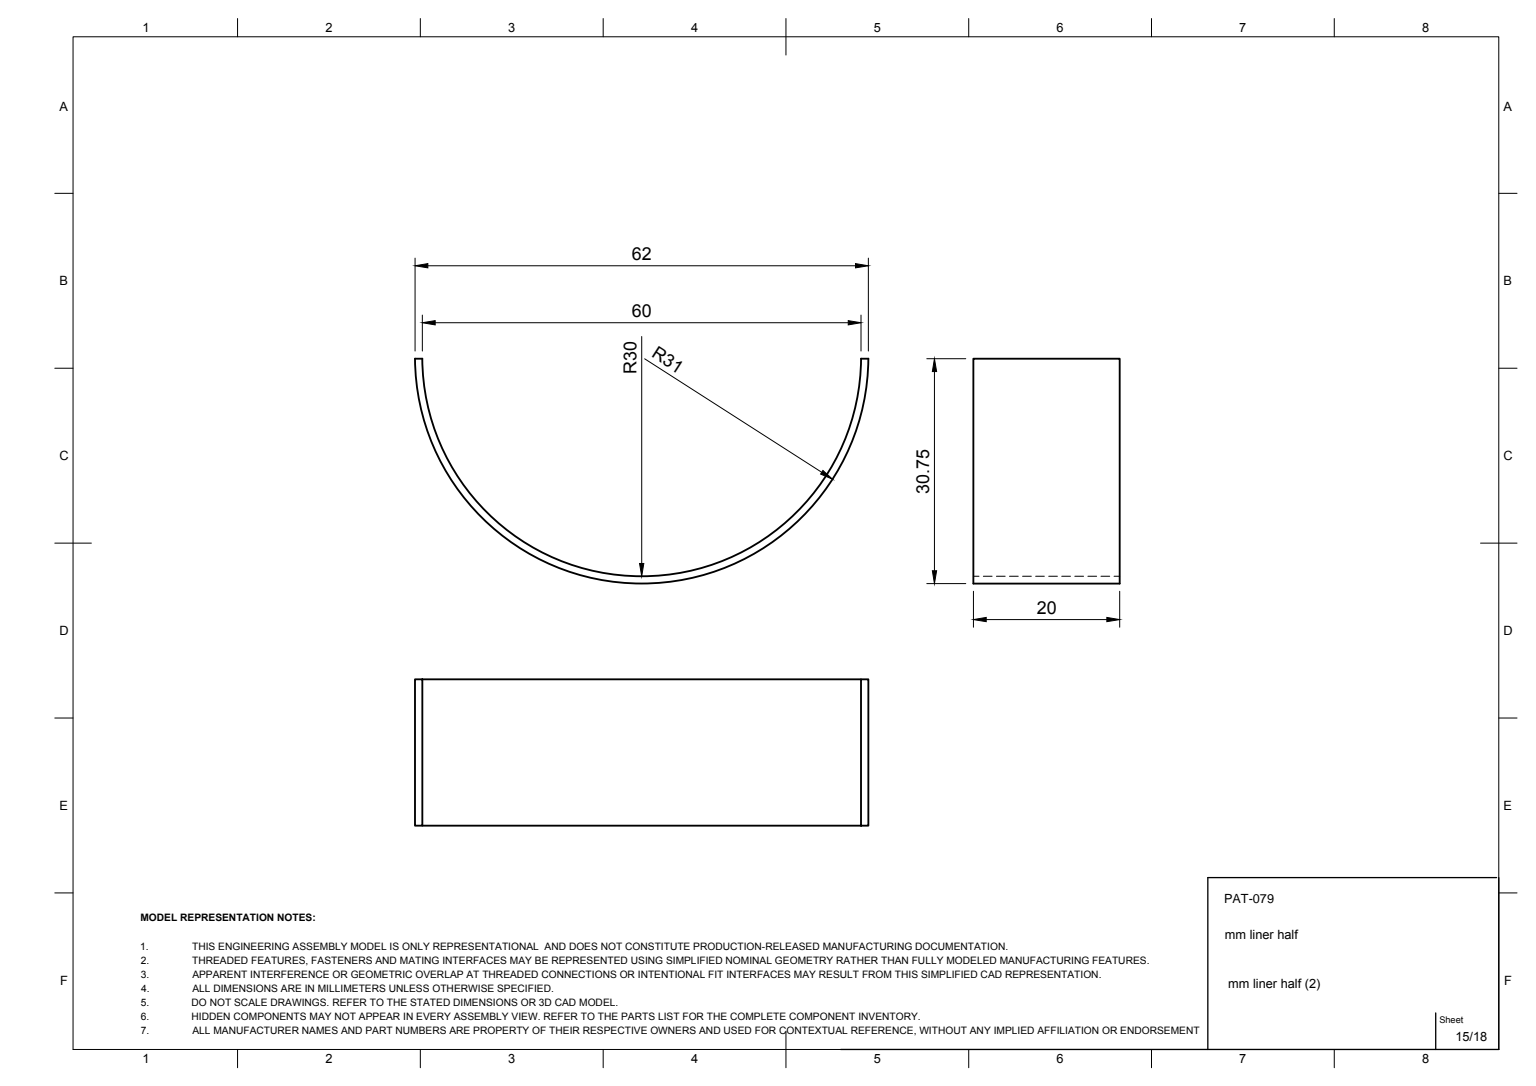
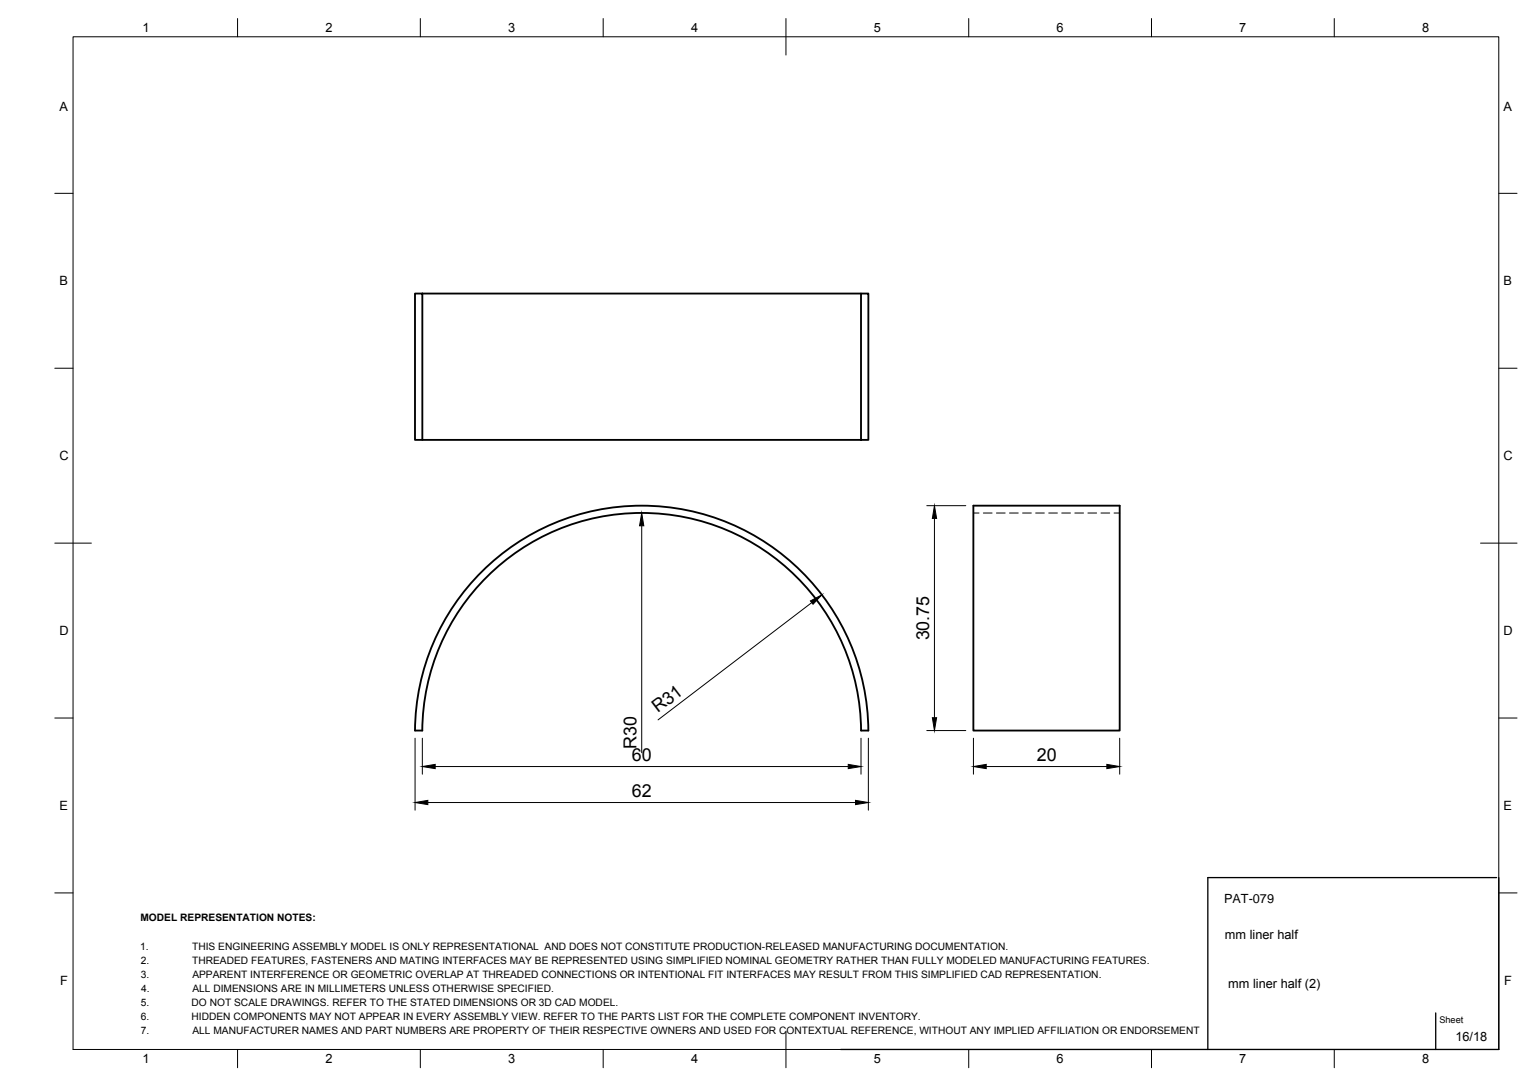
ISO-10303-21;
HEADER;
/* Generated by software containing ST-Developer
 * from STEP Tools, Inc. (www.steptools.com) 
 */

FILE_DESCRIPTION(
/* description */ ('Pipe clamp stand with threaded column'),
/* implementation_level */ '2;1');

FILE_NAME(
/* name */ 'mm liner half (2).step',
/* time_stamp */ '2026-10-27T10:55:48-07:00',
/* author */ (''),
/* organization */ (''),
/* preprocessor_version */ 'ST-DEVELOPER v20.2',
/* originating_system */ 'Autodesk Translation Framework v15.17.0.0',
/* authorisation */ '');

FILE_SCHEMA (('AUTOMOTIVE_DESIGN { 1 0 10303 214 3 1 1 }'));
ENDSEC;

DATA;
#10=MECHANICAL_DESIGN_GEOMETRIC_PRESENTATION_REPRESENTATION('',(#759),#34433);
#707=SHAPE_REPRESENTATION_RELATIONSHIP('SRR','None',#34549,#729);
#729=ADVANCED_BREP_SHAPE_REPRESENTATION('',(#789),#34417);
#759=STYLED_ITEM('',(#34736),#789);
#789=MANIFOLD_SOLID_BREP('Body1',#8786);
#959=PLANE('',#9474);
#960=PLANE('',#9475);
#961=PLANE('',#9476);
#962=PLANE('',#9483);
#1378=FACE_OUTER_BOUND('',#1908,.T.);
#1379=FACE_OUTER_BOUND('',#1909,.T.);
#1380=FACE_OUTER_BOUND('',#1910,.T.);
#1381=FACE_OUTER_BOUND('',#1911,.T.);
#1382=FACE_OUTER_BOUND('',#1912,.T.);
#1383=FACE_OUTER_BOUND('',#1913,.T.);
#1908=EDGE_LOOP('',(#7283,#7284,#7285,#7286));
#1909=EDGE_LOOP('',(#7287,#7288,#7289,#7290));
#1910=EDGE_LOOP('',(#7291,#7292,#7293,#7294));
#1911=EDGE_LOOP('',(#7295,#7296,#7297,#7298));
#1912=EDGE_LOOP('',(#7299,#7300,#7301,#7302));
#1913=EDGE_LOOP('',(#7303,#7304,#7305,#7306));
#2491=LINE('',#28574,#3108);
#2492=LINE('',#28576,#3109);
#2493=LINE('',#28578,#3110);
#2494=LINE('',#28579,#3111);
#2495=LINE('',#28583,#3112);
#2496=LINE('',#28585,#3113);
#2497=LINE('',#28587,#3114);
#2498=LINE('',#28588,#3115);
#3108=VECTOR('',#11004,1.);
#3109=VECTOR('',#11005,1.);
#3110=VECTOR('',#11006,1.);
#3111=VECTOR('',#11007,1.);
#3112=VECTOR('',#11010,1.);
#3113=VECTOR('',#11011,1.);
#3114=VECTOR('',#11012,1.);
#3115=VECTOR('',#11013,1.);
#3396=CIRCLE('',#9477,3.1);
#3397=CIRCLE('',#9478,3.);
#3398=CIRCLE('',#9480,3.);
#3399=CIRCLE('',#9482,3.1);
#4034=VERTEX_POINT('',#28572);
#4035=VERTEX_POINT('',#28573);
#4036=VERTEX_POINT('',#28575);
#4037=VERTEX_POINT('',#28577);
#4038=VERTEX_POINT('',#28581);
#4039=VERTEX_POINT('',#28582);
#4040=VERTEX_POINT('',#28584);
#4041=VERTEX_POINT('',#28586);
#5155=EDGE_CURVE('',#4034,#4035,#2491,.T.);
#5156=EDGE_CURVE('',#4036,#4034,#2492,.T.);
#5157=EDGE_CURVE('',#4037,#4036,#2493,.T.);
#5158=EDGE_CURVE('',#4035,#4037,#2494,.T.);
#5159=EDGE_CURVE('',#4038,#4039,#2495,.T.);
#5160=EDGE_CURVE('',#4040,#4038,#2496,.T.);
#5161=EDGE_CURVE('',#4041,#4040,#2497,.T.);
#5162=EDGE_CURVE('',#4039,#4041,#2498,.T.);
#5163=EDGE_CURVE('',#4035,#4038,#3396,.T.);
#5164=EDGE_CURVE('',#4040,#4037,#3397,.T.);
#5165=EDGE_CURVE('',#4041,#4036,#3398,.T.);
#5166=EDGE_CURVE('',#4034,#4039,#3399,.T.);
#7283=ORIENTED_EDGE('',*,*,#5155,.F.);
#7284=ORIENTED_EDGE('',*,*,#5156,.F.);
#7285=ORIENTED_EDGE('',*,*,#5157,.F.);
#7286=ORIENTED_EDGE('',*,*,#5158,.F.);
#7287=ORIENTED_EDGE('',*,*,#5159,.F.);
#7288=ORIENTED_EDGE('',*,*,#5160,.F.);
#7289=ORIENTED_EDGE('',*,*,#5161,.F.);
#7290=ORIENTED_EDGE('',*,*,#5162,.F.);
#7291=ORIENTED_EDGE('',*,*,#5160,.T.);
#7292=ORIENTED_EDGE('',*,*,#5163,.F.);
#7293=ORIENTED_EDGE('',*,*,#5158,.T.);
#7294=ORIENTED_EDGE('',*,*,#5164,.F.);
#7295=ORIENTED_EDGE('',*,*,#5161,.T.);
#7296=ORIENTED_EDGE('',*,*,#5164,.T.);
#7297=ORIENTED_EDGE('',*,*,#5157,.T.);
#7298=ORIENTED_EDGE('',*,*,#5165,.F.);
#7299=ORIENTED_EDGE('',*,*,#5159,.T.);
#7300=ORIENTED_EDGE('',*,*,#5166,.F.);
#7301=ORIENTED_EDGE('',*,*,#5155,.T.);
#7302=ORIENTED_EDGE('',*,*,#5163,.T.);
#7303=ORIENTED_EDGE('',*,*,#5162,.T.);
#7304=ORIENTED_EDGE('',*,*,#5165,.T.);
#7305=ORIENTED_EDGE('',*,*,#5156,.T.);
#7306=ORIENTED_EDGE('',*,*,#5166,.T.);
#8229=CYLINDRICAL_SURFACE('',#9479,3.);
#8230=CYLINDRICAL_SURFACE('',#9481,3.1);
#8615=ADVANCED_FACE('',(#1378),#959,.F.);
#8616=ADVANCED_FACE('',(#1379),#960,.F.);
#8617=ADVANCED_FACE('',(#1380),#961,.F.);
#8618=ADVANCED_FACE('',(#1381),#8229,.F.);
#8619=ADVANCED_FACE('',(#1382),#8230,.T.);
#8620=ADVANCED_FACE('',(#1383),#962,.T.);
#8786=CLOSED_SHELL('',(#8615,#8616,#8617,#8618,#8619,#8620));
#9473=AXIS2_PLACEMENT_3D('',#28570,#11000,#11001);
#9474=AXIS2_PLACEMENT_3D('',#28571,#11002,#11003);
#9475=AXIS2_PLACEMENT_3D('',#28580,#11008,#11009);
#9476=AXIS2_PLACEMENT_3D('',#28589,#11014,#11015);
#9477=AXIS2_PLACEMENT_3D('',#28590,#11016,#11017);
#9478=AXIS2_PLACEMENT_3D('',#28591,#11018,#11019);
#9479=AXIS2_PLACEMENT_3D('',#28592,#11020,#11021);
#9480=AXIS2_PLACEMENT_3D('',#28593,#11022,#11023);
#9481=AXIS2_PLACEMENT_3D('',#28594,#11024,#11025);
#9482=AXIS2_PLACEMENT_3D('',#28595,#11026,#11027);
#9483=AXIS2_PLACEMENT_3D('',#28596,#11028,#11029);
#11000=DIRECTION('axis',(0.,0.,1.));
#11001=DIRECTION('refdir',(1.,0.,0.));
#11002=DIRECTION('center_axis',(0.,0.,-1.));
#11003=DIRECTION('ref_axis',(-1.,0.,0.));
#11004=DIRECTION('',(0.,-1.,0.));
#11005=DIRECTION('',(1.,0.,0.));
#11006=DIRECTION('',(0.,1.,0.));
#11007=DIRECTION('',(-1.,0.,0.));
#11008=DIRECTION('center_axis',(0.,0.,-1.));
#11009=DIRECTION('ref_axis',(-1.,0.,0.));
#11010=DIRECTION('',(0.,1.,0.));
#11011=DIRECTION('',(-1.,0.,0.));
#11012=DIRECTION('',(0.,-1.,0.));
#11013=DIRECTION('',(1.,0.,0.));
#11014=DIRECTION('center_axis',(0.,1.,0.));
#11015=DIRECTION('ref_axis',(1.,0.,0.));
#11016=DIRECTION('center_axis',(0.,1.,0.));
#11017=DIRECTION('ref_axis',(1.,0.,0.));
#11018=DIRECTION('center_axis',(0.,-1.,0.));
#11019=DIRECTION('ref_axis',(1.,0.,0.));
#11020=DIRECTION('center_axis',(0.,1.,0.));
#11021=DIRECTION('ref_axis',(1.,0.,0.));
#11022=DIRECTION('center_axis',(0.,-1.,0.));
#11023=DIRECTION('ref_axis',(1.,0.,0.));
#11024=DIRECTION('center_axis',(0.,1.,0.));
#11025=DIRECTION('ref_axis',(1.,0.,0.));
#11026=DIRECTION('center_axis',(0.,1.,0.));
#11027=DIRECTION('ref_axis',(1.,0.,0.));
#11028=DIRECTION('center_axis',(0.,1.,0.));
#11029=DIRECTION('ref_axis',(1.,0.,0.));
#28570=CARTESIAN_POINT('',(0.,0.,0.));
#28571=CARTESIAN_POINT('Origin',(8.4,-1.1,27.975));
#28572=CARTESIAN_POINT('',(3.09989919190931,1.,27.975));
#28573=CARTESIAN_POINT('',(3.09989919190931,-1.,27.975));
#28574=CARTESIAN_POINT('',(3.09989919190931,-1.,27.975));
#28575=CARTESIAN_POINT('',(2.99989583152482,1.,27.975));
#28576=CARTESIAN_POINT('',(4.2,1.,27.975));
#28577=CARTESIAN_POINT('',(2.99989583152482,-1.,27.975));
#28578=CARTESIAN_POINT('',(2.99989583152482,-1.,27.975));
#28579=CARTESIAN_POINT('',(4.2,-1.,27.975));
#28580=CARTESIAN_POINT('Origin',(8.4,-1.1,27.975));
#28581=CARTESIAN_POINT('',(-3.09989919190931,-1.,27.975));
#28582=CARTESIAN_POINT('',(-3.09989919190931,1.,27.975));
#28583=CARTESIAN_POINT('',(-3.09989919190931,-1.,27.975));
#28584=CARTESIAN_POINT('',(-2.99989583152482,-1.,27.975));
#28585=CARTESIAN_POINT('',(4.2,-1.,27.975));
#28586=CARTESIAN_POINT('',(-2.99989583152482,1.,27.975));
#28587=CARTESIAN_POINT('',(-2.99989583152482,-1.,27.975));
#28588=CARTESIAN_POINT('',(4.2,1.,27.975));
#28589=CARTESIAN_POINT('Origin',(0.,-1.,28.));
#28590=CARTESIAN_POINT('Origin',(0.,-1.,28.));
#28591=CARTESIAN_POINT('Origin',(0.,-1.,28.));
#28592=CARTESIAN_POINT('Origin',(0.,-1.,28.));
#28593=CARTESIAN_POINT('Origin',(0.,1.,28.));
#28594=CARTESIAN_POINT('Origin',(0.,-1.,28.));
#28595=CARTESIAN_POINT('Origin',(0.,1.,28.));
#28596=CARTESIAN_POINT('Origin',(0.,1.,28.));
#34388=UNCERTAINTY_MEASURE_WITH_UNIT(LENGTH_MEASURE(0.001),#34434,
'DISTANCE_ACCURACY_VALUE',
'Maximum model space distance between geometric entities at asserted c
onnectivities');
#34404=UNCERTAINTY_MEASURE_WITH_UNIT(LENGTH_MEASURE(0.001),#34434,
'DISTANCE_ACCURACY_VALUE',
'Maximum model space distance between geometric entities at asserted c
onnectivities');
#34417=(
GEOMETRIC_REPRESENTATION_CONTEXT(3)
GLOBAL_UNCERTAINTY_ASSIGNED_CONTEXT((#34388))
GLOBAL_UNIT_ASSIGNED_CONTEXT((#34434,#34436,#34437))
REPRESENTATION_CONTEXT('','3D')
);
#34433=(
GEOMETRIC_REPRESENTATION_CONTEXT(3)
GLOBAL_UNCERTAINTY_ASSIGNED_CONTEXT((#34404))
GLOBAL_UNIT_ASSIGNED_CONTEXT((#34434,#34436,#34437))
REPRESENTATION_CONTEXT('','3D')
);
#34434=(
LENGTH_UNIT()
NAMED_UNIT(*)
SI_UNIT(.CENTI.,.METRE.)
);
#34436=(
NAMED_UNIT(*)
PLANE_ANGLE_UNIT()
SI_UNIT($,.RADIAN.)
);
#34437=(
NAMED_UNIT(*)
SI_UNIT($,.STERADIAN.)
SOLID_ANGLE_UNIT()
);
#34450=SHAPE_DEFINITION_REPRESENTATION(#34478,#34549);
#34478=PRODUCT_DEFINITION_SHAPE('',$,#34578);
#34549=SHAPE_REPRESENTATION('',(#9473),#34417);
#34565=PRODUCT_DEFINITION_CONTEXT('part definition',#34651,'design');
#34578=PRODUCT_DEFINITION('mm liner half (2)','mm liner half (2)',#34606,
#34565);
#34606=PRODUCT_DEFINITION_FORMATION('',$,#34665);
#34651=APPLICATION_CONTEXT(
'Core Data for Automotive Mechanical Design Process');
#34652=PRODUCT_CONTEXT('part definition',#34651,'mechanical');
#34665=PRODUCT('mm liner half (2)','mm liner half (2)','mm liner half (2)',(#34652));
#34730=COLOUR_RGB('Sky Blue',0.24,0.69,0.87);
#34731=FILL_AREA_STYLE_COLOUR('',#34730);
#34732=FILL_AREA_STYLE('',(#34731));
#34733=SURFACE_STYLE_FILL_AREA(#34732);
#34734=SURFACE_SIDE_STYLE('',(#34733));
#34735=SURFACE_STYLE_USAGE(.BOTH.,#34734);
#34736=PRESENTATION_STYLE_ASSIGNMENT((#34735));
ENDSEC;
END-ISO-10303-21;
